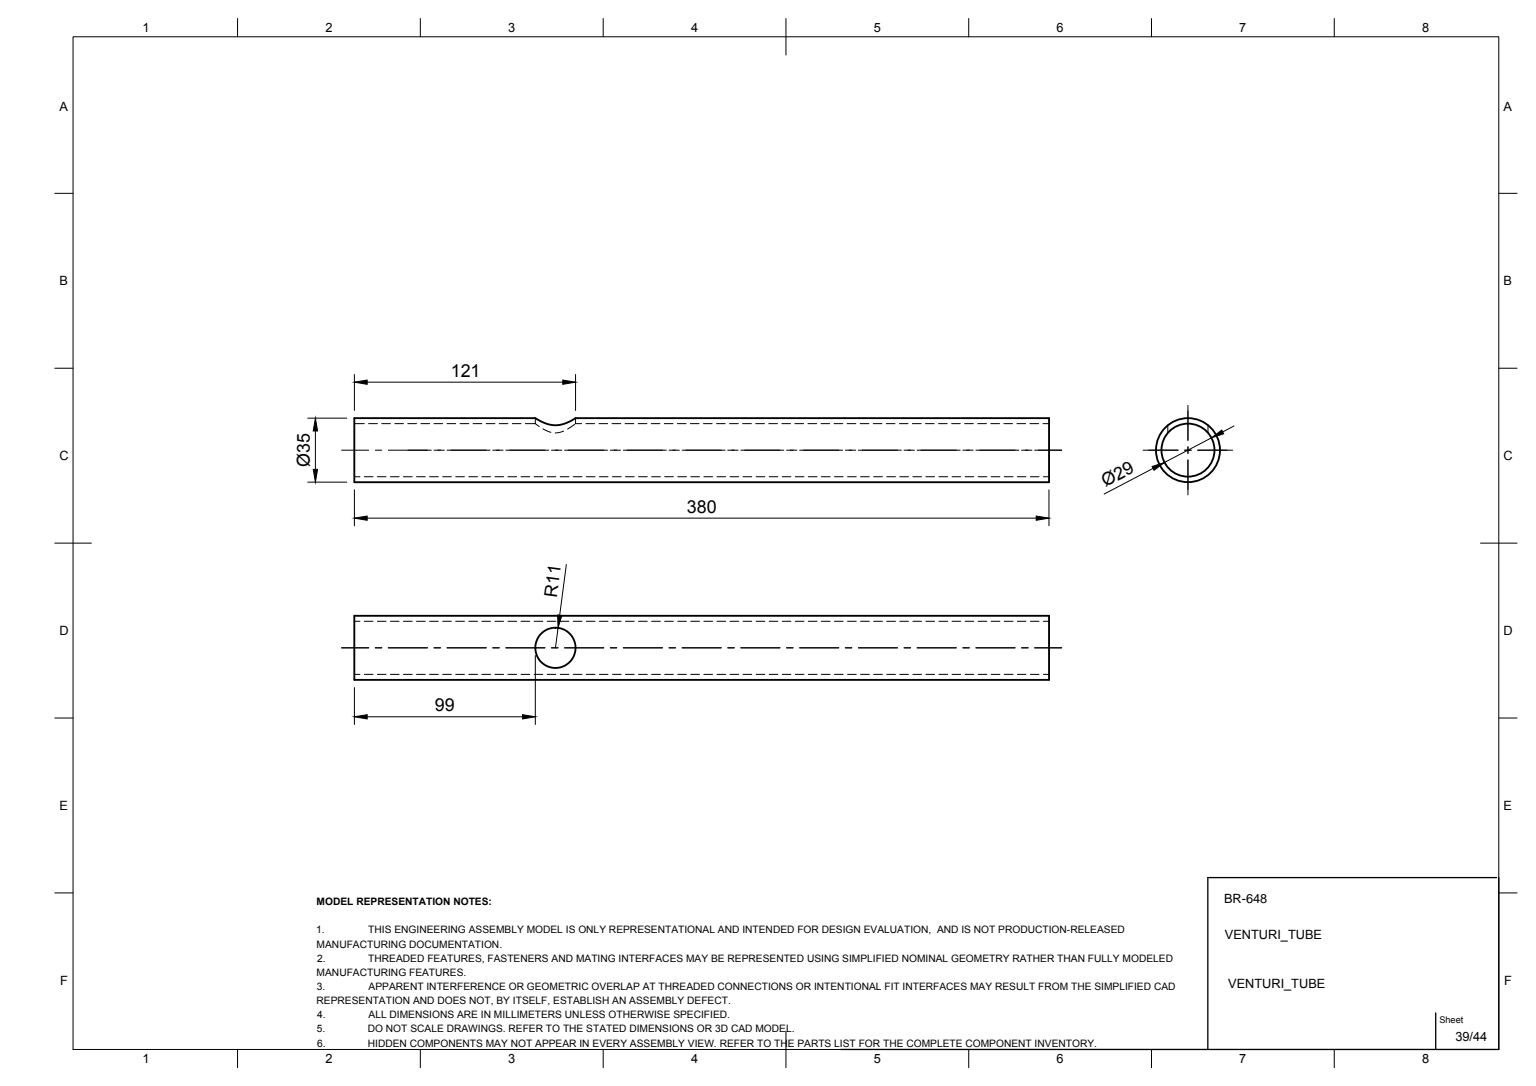
ISO-10303-21;
HEADER;
FILE_DESCRIPTION((''),'2;1');
FILE_NAME('VENTURI_TUBE.step','2026-10-01T22:05:39-07:00',(''),(''),'','','');
FILE_SCHEMA (('AUTOMOTIVE_DESIGN { 1 0 10303 214 3 1 1 }'));
ENDSEC;
DATA;
#10=MECHANICAL_DESIGN_GEOMETRIC_PRESENTATION_REPRESENTATION('',(#635),#24628);
#551=SHAPE_REPRESENTATION_RELATIONSHIP('SRR','None',#24825,#593) ;
#593=ADVANCED_BREP_SHAPE_REPRESENTATION('',(#674),#24615) ;
#635=STYLED_ITEM('',(#25034),#674) ;
#674=MANIFOLD_SOLID_BREP('VENTURI_TUBE',#13177) ;
#908=FACE_BOUND('',#4615,.T.) ;
#909=FACE_BOUND('',#4617,.T.) ;
#985=B_SPLINE_CURVE_WITH_KNOTS('',3,(#23796,#23797,#23798,#23799,#23800,
#23801,#23802,#23803,#23804,#23805,#23806,#23807,#23808,#23809),
 .UNSPECIFIED.,.F.,.F.,(4,2,2,2,2,2,4),(0.,0.222195827909919,0.444391655819838,
0.888783311639677,1.32318070684216,1.54037940444341,1.75757810204465),
 .UNSPECIFIED.) ;
#986=B_SPLINE_CURVE_WITH_KNOTS('',3,(#23811,#23812,#23813,#23814,#23815,
#23816,#23817,#23818,#23819,#23820,#23821,#23822,#23823,#23824),
 .UNSPECIFIED.,.F.,.F.,(4,2,2,2,2,2,4),(5.27273430613395,5.48993300373519,
5.70713170133643,6.14152909653892,6.58592075235876,6.80811658026868,7.0303124081786),
 .UNSPECIFIED.) ;
#987=B_SPLINE_CURVE_WITH_KNOTS('',3,(#23828,#23829,#23830,#23831,#23832,
#23833,#23834,#23835,#23836,#23837,#23838,#23839,#23840,#23841),
 .UNSPECIFIED.,.F.,.F.,(4,2,2,2,2,2,4),(0.,0.215433509152083,0.430867018304165,
0.86173403660833,1.28909704518263,1.50277854946978,1.71646005375693),
 .UNSPECIFIED.) ;
#988=B_SPLINE_CURVE_WITH_KNOTS('',3,(#23843,#23844,#23845,#23846,#23847,
#23848,#23849,#23850,#23851,#23852,#23853,#23854,#23855,#23856),
 .UNSPECIFIED.,.F.,.F.,(4,2,2,2,2,2,4),(5.14938016127078,5.36306166555793,
5.57674316984508,6.00410617841938,6.43497319672355,6.65040670587563,6.86584021502771),
 .UNSPECIFIED.) ;
#989=B_SPLINE_CURVE_WITH_KNOTS('',3,(#23857,#23858,#23859,#23860,#23861,
#23862,#23863,#23864,#23865,#23866,#23867,#23868,#23869,#23870,#23871,#23872,
#23873,#23874,#23875,#23876,#23877,#23878,#23879,#23880,#23881,#23882),
 .UNSPECIFIED.,.F.,.F.,(4,2,2,2,2,2,2,2,2,2,2,2,4),(1.71646005375693,1.93014155804408,
2.14382306233123,2.57118607090553,3.00205308920969,3.21748659836177,3.43292010751385,
3.64835361666594,3.86378712581802,4.29465414412218,4.72201715269648,4.93569865698363,
5.14938016127078),.UNSPECIFIED.) ;
#990=B_SPLINE_CURVE_WITH_KNOTS('',3,(#23883,#23884,#23885,#23886,#23887,
#23888,#23889,#23890,#23891,#23892,#23893,#23894,#23895,#23896,#23897,#23898,
#23899,#23900,#23901,#23902,#23903,#23904,#23905,#23906,#23907,#23908),
 .UNSPECIFIED.,.F.,.F.,(4,2,2,2,2,2,2,2,2,2,2,2,4),(1.75757810204465,1.97477679964589,
2.19197549724714,2.62637289244962,3.07076454826946,3.29296037617938,3.5151562040893,
3.73735203199922,3.95954785990914,4.40393951572897,4.83833691093146,5.0555356085327,
5.27273430613395),.UNSPECIFIED.) ;
#1707=LINE('',#23826,#2543) ;
#1708=LINE('',#23912,#2544) ;
#1709=LINE('',#23914,#2545) ;
#1710=LINE('',#23919,#2546) ;
#1711=LINE('',#23921,#2547) ;
#2543=VECTOR('',#19160,1.1) ;
#2544=VECTOR('',#19165,1.45) ;
#2545=VECTOR('',#19166,1.45) ;
#2546=VECTOR('',#19173,1.75) ;
#2547=VECTOR('',#19174,1.75) ;
#2917=CYLINDRICAL_SURFACE('',#15183,1.1) ;
#2918=CYLINDRICAL_SURFACE('',#15184,1.45) ;
#2919=CYLINDRICAL_SURFACE('',#15187,1.75) ;
#3622=FACE_OUTER_BOUND('',#4611,.T.) ;
#3623=FACE_OUTER_BOUND('',#4612,.T.) ;
#3624=FACE_OUTER_BOUND('',#4613,.T.) ;
#3625=FACE_OUTER_BOUND('',#4614,.T.) ;
#3626=FACE_OUTER_BOUND('',#4616,.T.) ;
#4611=EDGE_LOOP('',(#11567,#11568,#11569,#11570,#11571,#11572,#11573,#11574)) ;
#4612=EDGE_LOOP('',(#11575,#11576,#11577,#11578,#11579,#11580,#11581,#11582,
#11583)) ;
#4613=EDGE_LOOP('',(#11584,#11585,#11586,#11587,#11588,#11589,#11590,#11591,
#11592)) ;
#4614=EDGE_LOOP('',(#11593)) ;
#4615=EDGE_LOOP('',(#11594)) ;
#4616=EDGE_LOOP('',(#11595)) ;
#4617=EDGE_LOOP('',(#11596)) ;
#5469=CIRCLE('',#15185,1.45) ;
#5470=CIRCLE('',#15186,1.45) ;
#5471=CIRCLE('',#15188,1.75) ;
#5472=CIRCLE('',#15189,1.75) ;
#6591=VERTEX_POINT('',#23794) ;
#6592=VERTEX_POINT('',#23795) ;
#6593=VERTEX_POINT('',#23810) ;
#6594=VERTEX_POINT('',#23825) ;
#6595=VERTEX_POINT('',#23827) ;
#6596=VERTEX_POINT('',#23842) ;
#6597=VERTEX_POINT('',#23910) ;
#6598=VERTEX_POINT('',#23913) ;
#6599=VERTEX_POINT('',#23917) ;
#6600=VERTEX_POINT('',#23920) ;
#8273=EDGE_CURVE('',#6591,#6592,#985,.T.) ;
#8274=EDGE_CURVE('',#6593,#6591,#986,.T.) ;
#8275=EDGE_CURVE('',#6593,#6594,#1707,.T.) ;
#8276=EDGE_CURVE('',#6595,#6594,#987,.T.) ;
#8277=EDGE_CURVE('',#6596,#6595,#988,.T.) ;
#8278=EDGE_CURVE('',#6594,#6596,#989,.T.) ;
#8279=EDGE_CURVE('',#6592,#6593,#990,.T.) ;
#8280=EDGE_CURVE('',#6597,#6597,#5469,.T.) ;
#8281=EDGE_CURVE('',#6597,#6593,#1708,.T.) ;
#8282=EDGE_CURVE('',#6592,#6598,#1709,.T.) ;
#8283=EDGE_CURVE('',#6598,#6598,#5470,.T.) ;
#8284=EDGE_CURVE('',#6599,#6599,#5471,.T.) ;
#8285=EDGE_CURVE('',#6599,#6596,#1710,.T.) ;
#8286=EDGE_CURVE('',#6594,#6600,#1711,.T.) ;
#8287=EDGE_CURVE('',#6600,#6600,#5472,.T.) ;
#11567=ORIENTED_EDGE('',*,*,#8273,.F.) ;
#11568=ORIENTED_EDGE('',*,*,#8274,.F.) ;
#11569=ORIENTED_EDGE('',*,*,#8275,.T.) ;
#11570=ORIENTED_EDGE('',*,*,#8276,.F.) ;
#11571=ORIENTED_EDGE('',*,*,#8277,.F.) ;
#11572=ORIENTED_EDGE('',*,*,#8278,.F.) ;
#11573=ORIENTED_EDGE('',*,*,#8275,.F.) ;
#11574=ORIENTED_EDGE('',*,*,#8279,.F.) ;
#11575=ORIENTED_EDGE('',*,*,#8280,.F.) ;
#11576=ORIENTED_EDGE('',*,*,#8281,.T.) ;
#11577=ORIENTED_EDGE('',*,*,#8274,.T.) ;
#11578=ORIENTED_EDGE('',*,*,#8273,.T.) ;
#11579=ORIENTED_EDGE('',*,*,#8282,.T.) ;
#11580=ORIENTED_EDGE('',*,*,#8283,.F.) ;
#11581=ORIENTED_EDGE('',*,*,#8282,.F.) ;
#11582=ORIENTED_EDGE('',*,*,#8279,.T.) ;
#11583=ORIENTED_EDGE('',*,*,#8281,.F.) ;
#11584=ORIENTED_EDGE('',*,*,#8284,.F.) ;
#11585=ORIENTED_EDGE('',*,*,#8285,.T.) ;
#11586=ORIENTED_EDGE('',*,*,#8277,.T.) ;
#11587=ORIENTED_EDGE('',*,*,#8276,.T.) ;
#11588=ORIENTED_EDGE('',*,*,#8286,.T.) ;
#11589=ORIENTED_EDGE('',*,*,#8287,.F.) ;
#11590=ORIENTED_EDGE('',*,*,#8286,.F.) ;
#11591=ORIENTED_EDGE('',*,*,#8278,.T.) ;
#11592=ORIENTED_EDGE('',*,*,#8285,.F.) ;
#11593=ORIENTED_EDGE('',*,*,#8287,.T.) ;
#11594=ORIENTED_EDGE('',*,*,#8280,.T.) ;
#11595=ORIENTED_EDGE('',*,*,#8284,.T.) ;
#11596=ORIENTED_EDGE('',*,*,#8283,.T.) ;
#12287=PLANE('',#15190) ;
#12288=PLANE('',#15191) ;
#13017=ADVANCED_FACE('',(#3622),#2917,.F.) ;
#13018=ADVANCED_FACE('',(#3623),#2918,.F.) ;
#13019=ADVANCED_FACE('',(#3624),#2919,.T.) ;
#13020=ADVANCED_FACE('',(#3625,#908),#12287,.T.) ;
#13021=ADVANCED_FACE('',(#3626,#909),#12288,.T.) ;
#13177=CLOSED_SHELL('',(#13017,#13018,#13019,#13020,#13021)) ;
#15182=AXIS2_PLACEMENT_3D('',#23792,#19156,#19157) ;
#15183=AXIS2_PLACEMENT_3D('',#23793,#19158,#19159) ;
#15184=AXIS2_PLACEMENT_3D('',#23909,#19161,#19162) ;
#15185=AXIS2_PLACEMENT_3D('',#23911,#19163,#19164) ;
#15186=AXIS2_PLACEMENT_3D('',#23915,#19167,#19168) ;
#15187=AXIS2_PLACEMENT_3D('',#23916,#19169,#19170) ;
#15188=AXIS2_PLACEMENT_3D('',#23918,#19171,#19172) ;
#15189=AXIS2_PLACEMENT_3D('',#23922,#19175,#19176) ;
#15190=AXIS2_PLACEMENT_3D('',#23923,#19177,#19178) ;
#15191=AXIS2_PLACEMENT_3D('',#23924,#19179,#19180) ;
#19156=DIRECTION('axis',(0.,0.,1.)) ;
#19157=DIRECTION('refdir',(1.,0.,0.)) ;
#19158=DIRECTION('center_axis',(0.,0.,1.)) ;
#19159=DIRECTION('ref_axis',(1.,0.,0.)) ;
#19160=DIRECTION('',(0.,0.,1.)) ;
#19161=DIRECTION('center_axis',(1.,0.,0.)) ;
#19162=DIRECTION('ref_axis',(0.,0.,-1.)) ;
#19163=DIRECTION('center_axis',(1.,0.,0.)) ;
#19164=DIRECTION('ref_axis',(0.,0.,-1.)) ;
#19165=DIRECTION('',(1.,0.,0.)) ;
#19166=DIRECTION('',(1.,0.,0.)) ;
#19167=DIRECTION('center_axis',(-1.,0.,0.)) ;
#19168=DIRECTION('ref_axis',(0.,0.,-1.)) ;
#19169=DIRECTION('center_axis',(1.,0.,0.)) ;
#19170=DIRECTION('ref_axis',(0.,0.,-1.)) ;
#19171=DIRECTION('center_axis',(1.,0.,0.)) ;
#19172=DIRECTION('ref_axis',(0.,0.,-1.)) ;
#19173=DIRECTION('',(-1.,0.,0.)) ;
#19174=DIRECTION('',(-1.,0.,0.)) ;
#19175=DIRECTION('center_axis',(-1.,0.,0.)) ;
#19176=DIRECTION('ref_axis',(0.,0.,-1.)) ;
#19177=DIRECTION('center_axis',(-1.,0.,0.)) ;
#19178=DIRECTION('ref_axis',(0.,0.,1.)) ;
#19179=DIRECTION('center_axis',(1.,0.,0.)) ;
#19180=DIRECTION('ref_axis',(0.,0.,-1.)) ;
#23792=CARTESIAN_POINT('',(0.,0.,0.)) ;
#23793=CARTESIAN_POINT('Origin',(-3.,-1.8,-15.55)) ;
#23794=CARTESIAN_POINT('',(-3.,-2.9,-15.5552778186154)) ;
#23795=CARTESIAN_POINT('',(-1.9,-1.8,-15.05)) ;
#23796=CARTESIAN_POINT('Ctrl Pts',(-3.,-2.9,-15.5552778186154)) ;
#23797=CARTESIAN_POINT('Ctrl Pts',(-2.92593472403003,-2.9,-15.5552778186154)) ;
#23798=CARTESIAN_POINT('Ctrl Pts',(-2.85172404139738,-2.89244970013866,
-15.5463012974331)) ;
#23799=CARTESIAN_POINT('Ctrl Pts',(-2.70730976928893,-2.86290382536062,
-15.5134793386501)) ;
#23800=CARTESIAN_POINT('Ctrl Pts',(-2.6370687680745,-2.84092482077356,-15.4897837774916)) ;
#23801=CARTESIAN_POINT('Ctrl Pts',(-2.43708115985337,-2.75608431930036,
-15.4070006970031)) ;
#23802=CARTESIAN_POINT('Ctrl Pts',(-2.31772068603768,-2.67335560464808,
-15.3370016719564)) ;
#23803=CARTESIAN_POINT('Ctrl Pts',(-2.12879302508191,-2.48442794369232,
-15.2169163796472)) ;
#23804=CARTESIAN_POINT('Ctrl Pts',(-2.04479613304032,-2.36484101063073,
-15.1570971235734)) ;
#23805=CARTESIAN_POINT('Ctrl Pts',(-1.95889743356179,-2.16258851937244,
-15.0942927158064)) ;
#23806=CARTESIAN_POINT('Ctrl Pts',(-1.93671733228809,-2.09139288005492,
-15.0776864580625)) ;
#23807=CARTESIAN_POINT('Ctrl Pts',(-1.90726216861058,-1.94630062852708,
-15.0555340958438)) ;
#23808=CARTESIAN_POINT('Ctrl Pts',(-1.9,-1.87239956586708,-15.05)) ;
#23809=CARTESIAN_POINT('Ctrl Pts',(-1.9,-1.8,-15.05)) ;
#23810=CARTESIAN_POINT('',(-4.1,-1.8,-15.05)) ;
#23811=CARTESIAN_POINT('Ctrl Pts',(-4.1,-1.8,-15.05)) ;
#23812=CARTESIAN_POINT('Ctrl Pts',(-4.1,-1.87239956586708,-15.05)) ;
#23813=CARTESIAN_POINT('Ctrl Pts',(-4.09273783138942,-1.94630062852708,
-15.0555340958438)) ;
#23814=CARTESIAN_POINT('Ctrl Pts',(-4.06328266771191,-2.09139288005492,
-15.0776864580625)) ;
#23815=CARTESIAN_POINT('Ctrl Pts',(-4.04110256643821,-2.16258851937244,
-15.0942927158064)) ;
#23816=CARTESIAN_POINT('Ctrl Pts',(-3.95520386695968,-2.36484101063073,
-15.1570971235734)) ;
#23817=CARTESIAN_POINT('Ctrl Pts',(-3.87120697491809,-2.48442794369232,
-15.2169163796472)) ;
#23818=CARTESIAN_POINT('Ctrl Pts',(-3.68227931396233,-2.67335560464808,
-15.3370016719564)) ;
#23819=CARTESIAN_POINT('Ctrl Pts',(-3.56291884014663,-2.75608431930036,
-15.4070006970031)) ;
#23820=CARTESIAN_POINT('Ctrl Pts',(-3.3629312319255,-2.84092482077356,-15.4897837774916)) ;
#23821=CARTESIAN_POINT('Ctrl Pts',(-3.29269023071107,-2.86290382536062,
-15.5134793386501)) ;
#23822=CARTESIAN_POINT('Ctrl Pts',(-3.14827595860262,-2.89244970013866,
-15.5463012974331)) ;
#23823=CARTESIAN_POINT('Ctrl Pts',(-3.07406527596997,-2.9,-15.5552778186154)) ;
#23824=CARTESIAN_POINT('Ctrl Pts',(-3.,-2.9,-15.5552778186154)) ;
#23825=CARTESIAN_POINT('',(-4.1,-1.8,-14.75)) ;
#23826=CARTESIAN_POINT('',(-4.1,-1.8,-15.55)) ;
#23827=CARTESIAN_POINT('',(-3.,-2.9,-15.1389342411184)) ;
#23828=CARTESIAN_POINT('Ctrl Pts',(-3.,-2.9,-15.1389342411184)) ;
#23829=CARTESIAN_POINT('Ctrl Pts',(-3.07181116971736,-2.9,-15.1389342411184)) ;
#23830=CARTESIAN_POINT('Ctrl Pts',(-3.14499752680644,-2.89286661726534,
-15.1330764609861)) ;
#23831=CARTESIAN_POINT('Ctrl Pts',(-3.28883700701042,-2.86393369738317,
-15.1104380225034)) ;
#23832=CARTESIAN_POINT('Ctrl Pts',(-3.3595029893093,-2.84215035317734,-15.0937184190741)) ;
#23833=CARTESIAN_POINT('Ctrl Pts',(-3.56118090687537,-2.75726493295417,
-15.0333835136228)) ;
#23834=CARTESIAN_POINT('Ctrl Pts',(-3.68198795957211,-2.6736469590383,-14.9799062284422)) ;
#23835=CARTESIAN_POINT('Ctrl Pts',(-3.87286762925623,-2.48276728935417,
-14.8851973706734)) ;
#23836=CARTESIAN_POINT('Ctrl Pts',(-3.95701740777658,-2.36176319521959,
-14.8367787014793)) ;
#23837=CARTESIAN_POINT('Ctrl Pts',(-4.0422651124962,-2.15923323536895,-14.7858537872249)) ;
#23838=CARTESIAN_POINT('Ctrl Pts',(-4.06409704750744,-2.08825332179439,
-14.7723789472322)) ;
#23839=CARTESIAN_POINT('Ctrl Pts',(-4.09297019244892,-1.9442520796829,-14.7544468449727)) ;
#23840=CARTESIAN_POINT('Ctrl Pts',(-4.1,-1.87122716809572,-14.75)) ;
#23841=CARTESIAN_POINT('Ctrl Pts',(-4.1,-1.8,-14.75)) ;
#23842=CARTESIAN_POINT('',(-1.9,-1.8,-14.75)) ;
#23843=CARTESIAN_POINT('Ctrl Pts',(-1.9,-1.8,-14.75)) ;
#23844=CARTESIAN_POINT('Ctrl Pts',(-1.9,-1.87122716809572,-14.75)) ;
#23845=CARTESIAN_POINT('Ctrl Pts',(-1.90702980755108,-1.9442520796829,-14.7544468449727)) ;
#23846=CARTESIAN_POINT('Ctrl Pts',(-1.93590295249256,-2.08825332179439,
-14.7723789472322)) ;
#23847=CARTESIAN_POINT('Ctrl Pts',(-1.9577348875038,-2.15923323536894,-14.7858537872249)) ;
#23848=CARTESIAN_POINT('Ctrl Pts',(-2.04298259222342,-2.36176319521959,
-14.8367787014793)) ;
#23849=CARTESIAN_POINT('Ctrl Pts',(-2.12713237074377,-2.48276728935417,
-14.8851973706734)) ;
#23850=CARTESIAN_POINT('Ctrl Pts',(-2.31801204042789,-2.6736469590383,-14.9799062284422)) ;
#23851=CARTESIAN_POINT('Ctrl Pts',(-2.43881909312463,-2.75726493295417,
-15.0333835136228)) ;
#23852=CARTESIAN_POINT('Ctrl Pts',(-2.6404970106907,-2.84215035317734,-15.0937184190741)) ;
#23853=CARTESIAN_POINT('Ctrl Pts',(-2.71116299298958,-2.86393369738317,
-15.1104380225034)) ;
#23854=CARTESIAN_POINT('Ctrl Pts',(-2.85500247319356,-2.89286661726534,
-15.1330764609861)) ;
#23855=CARTESIAN_POINT('Ctrl Pts',(-2.92818883028264,-2.9,-15.1389342411184)) ;
#23856=CARTESIAN_POINT('Ctrl Pts',(-3.,-2.9,-15.1389342411184)) ;
#23857=CARTESIAN_POINT('Ctrl Pts',(-4.1,-1.8,-14.75)) ;
#23858=CARTESIAN_POINT('Ctrl Pts',(-4.1,-1.72877283190428,-14.75)) ;
#23859=CARTESIAN_POINT('Ctrl Pts',(-4.09297019244892,-1.6557479203171,-14.7544468449727)) ;
#23860=CARTESIAN_POINT('Ctrl Pts',(-4.06409704750744,-1.51174667820561,
-14.7723789472322)) ;
#23861=CARTESIAN_POINT('Ctrl Pts',(-4.0422651124962,-1.44076676463106,-14.7858537872249)) ;
#23862=CARTESIAN_POINT('Ctrl Pts',(-3.95701740777658,-1.23823680478041,
-14.8367787014793)) ;
#23863=CARTESIAN_POINT('Ctrl Pts',(-3.87286762925623,-1.11723271064583,
-14.8851973706734)) ;
#23864=CARTESIAN_POINT('Ctrl Pts',(-3.68198795957211,-0.926353040961702,
-14.9799062284422)) ;
#23865=CARTESIAN_POINT('Ctrl Pts',(-3.56118090687537,-0.842735067045828,
-15.0333835136228)) ;
#23866=CARTESIAN_POINT('Ctrl Pts',(-3.3595029893093,-0.757849646822659,
-15.0937184190741)) ;
#23867=CARTESIAN_POINT('Ctrl Pts',(-3.28883700701042,-0.736066302616833,
-15.1104380225034)) ;
#23868=CARTESIAN_POINT('Ctrl Pts',(-3.14499752680644,-0.707133382734658,
-15.1330764609861)) ;
#23869=CARTESIAN_POINT('Ctrl Pts',(-3.07181116971736,-0.7,-15.1389342411184)) ;
#23870=CARTESIAN_POINT('Ctrl Pts',(-2.92818883028264,-0.7,-15.1389342411184)) ;
#23871=CARTESIAN_POINT('Ctrl Pts',(-2.85500247319356,-0.707133382734658,
-15.1330764609861)) ;
#23872=CARTESIAN_POINT('Ctrl Pts',(-2.71116299298958,-0.736066302616833,
-15.1104380225034)) ;
#23873=CARTESIAN_POINT('Ctrl Pts',(-2.6404970106907,-0.75784964682266,-15.0937184190741)) ;
#23874=CARTESIAN_POINT('Ctrl Pts',(-2.43881909312463,-0.842735067045828,
-15.0333835136228)) ;
#23875=CARTESIAN_POINT('Ctrl Pts',(-2.31801204042789,-0.926353040961702,
-14.9799062284422)) ;
#23876=CARTESIAN_POINT('Ctrl Pts',(-2.12713237074376,-1.11723271064583,
-14.8851973706734)) ;
#23877=CARTESIAN_POINT('Ctrl Pts',(-2.04298259222342,-1.23823680478041,
-14.8367787014793)) ;
#23878=CARTESIAN_POINT('Ctrl Pts',(-1.9577348875038,-1.44076676463106,-14.7858537872249)) ;
#23879=CARTESIAN_POINT('Ctrl Pts',(-1.93590295249256,-1.51174667820561,
-14.7723789472322)) ;
#23880=CARTESIAN_POINT('Ctrl Pts',(-1.90702980755108,-1.6557479203171,-14.7544468449727)) ;
#23881=CARTESIAN_POINT('Ctrl Pts',(-1.9,-1.72877283190428,-14.75)) ;
#23882=CARTESIAN_POINT('Ctrl Pts',(-1.9,-1.8,-14.75)) ;
#23883=CARTESIAN_POINT('Ctrl Pts',(-1.9,-1.8,-15.05)) ;
#23884=CARTESIAN_POINT('Ctrl Pts',(-1.9,-1.72760043413292,-15.05)) ;
#23885=CARTESIAN_POINT('Ctrl Pts',(-1.90726216861058,-1.65369937147292,
-15.0555340958438)) ;
#23886=CARTESIAN_POINT('Ctrl Pts',(-1.93671733228809,-1.50860711994508,
-15.0776864580625)) ;
#23887=CARTESIAN_POINT('Ctrl Pts',(-1.95889743356178,-1.43741148062756,
-15.0942927158064)) ;
#23888=CARTESIAN_POINT('Ctrl Pts',(-2.04479613304032,-1.23515898936927,
-15.1570971235734)) ;
#23889=CARTESIAN_POINT('Ctrl Pts',(-2.12879302508191,-1.11557205630768,
-15.2169163796472)) ;
#23890=CARTESIAN_POINT('Ctrl Pts',(-2.31772068603768,-0.92664439535192,
-15.3370016719564)) ;
#23891=CARTESIAN_POINT('Ctrl Pts',(-2.43708115985337,-0.843915680699641,
-15.4070006970031)) ;
#23892=CARTESIAN_POINT('Ctrl Pts',(-2.6370687680745,-0.759075179226438,
-15.4897837774916)) ;
#23893=CARTESIAN_POINT('Ctrl Pts',(-2.70730976928893,-0.737096174639381,
-15.5134793386501)) ;
#23894=CARTESIAN_POINT('Ctrl Pts',(-2.85172404139738,-0.707550299861341,
-15.5463012974331)) ;
#23895=CARTESIAN_POINT('Ctrl Pts',(-2.92593472403003,-0.7,-15.5552778186154)) ;
#23896=CARTESIAN_POINT('Ctrl Pts',(-3.07406527596997,-0.7,-15.5552778186154)) ;
#23897=CARTESIAN_POINT('Ctrl Pts',(-3.14827595860262,-0.707550299861341,
-15.5463012974331)) ;
#23898=CARTESIAN_POINT('Ctrl Pts',(-3.29269023071107,-0.737096174639381,
-15.5134793386501)) ;
#23899=CARTESIAN_POINT('Ctrl Pts',(-3.3629312319255,-0.759075179226438,
-15.4897837774916)) ;
#23900=CARTESIAN_POINT('Ctrl Pts',(-3.56291884014663,-0.843915680699641,
-15.4070006970031)) ;
#23901=CARTESIAN_POINT('Ctrl Pts',(-3.68227931396233,-0.92664439535192,
-15.3370016719564)) ;
#23902=CARTESIAN_POINT('Ctrl Pts',(-3.87120697491809,-1.11557205630768,
-15.2169163796472)) ;
#23903=CARTESIAN_POINT('Ctrl Pts',(-3.95520386695968,-1.23515898936927,
-15.1570971235734)) ;
#23904=CARTESIAN_POINT('Ctrl Pts',(-4.04110256643821,-1.43741148062756,
-15.0942927158064)) ;
#23905=CARTESIAN_POINT('Ctrl Pts',(-4.06328266771191,-1.50860711994508,
-15.0776864580625)) ;
#23906=CARTESIAN_POINT('Ctrl Pts',(-4.09273783138942,-1.65369937147292,
-15.0555340958438)) ;
#23907=CARTESIAN_POINT('Ctrl Pts',(-4.1,-1.72760043413292,-15.05)) ;
#23908=CARTESIAN_POINT('Ctrl Pts',(-4.1,-1.8,-15.05)) ;
#23909=CARTESIAN_POINT('Origin',(-11.,-1.8,-16.5)) ;
#23910=CARTESIAN_POINT('',(-30.,-1.8,-15.05)) ;
#23911=CARTESIAN_POINT('Origin',(-30.,-1.8,-16.5)) ;
#23912=CARTESIAN_POINT('',(-11.,-1.8,-15.05)) ;
#23913=CARTESIAN_POINT('',(8.,-1.8,-15.05)) ;
#23914=CARTESIAN_POINT('',(-11.,-1.8,-15.05)) ;
#23915=CARTESIAN_POINT('Origin',(8.,-1.8,-16.5)) ;
#23916=CARTESIAN_POINT('Origin',(-11.,-1.8,-16.5)) ;
#23917=CARTESIAN_POINT('',(8.,-1.8,-14.75)) ;
#23918=CARTESIAN_POINT('Origin',(8.,-1.8,-16.5)) ;
#23919=CARTESIAN_POINT('',(-11.,-1.8,-14.75)) ;
#23920=CARTESIAN_POINT('',(-30.,-1.8,-14.75)) ;
#23921=CARTESIAN_POINT('',(-11.,-1.8,-14.75)) ;
#23922=CARTESIAN_POINT('Origin',(-30.,-1.8,-16.5)) ;
#23923=CARTESIAN_POINT('Origin',(-30.,-1.8,-16.5)) ;
#23924=CARTESIAN_POINT('Origin',(8.,-1.8,-16.5)) ;
#24567=UNCERTAINTY_MEASURE_WITH_UNIT(LENGTH_MEASURE(0.001),#24629,
'DISTANCE_ACCURACY_VALUE',
'Maximum model space distance between geometric entities at asserted c
onnectivities') ;
#24580=UNCERTAINTY_MEASURE_WITH_UNIT(LENGTH_MEASURE(0.001),#24629,
'DISTANCE_ACCURACY_VALUE',
'Maximum model space distance between geometric entities at asserted c
onnectivities') ;
#24615=(
GEOMETRIC_REPRESENTATION_CONTEXT(3)
GLOBAL_UNCERTAINTY_ASSIGNED_CONTEXT((#24567))
GLOBAL_UNIT_ASSIGNED_CONTEXT((#24629,#24631,#24632))
REPRESENTATION_CONTEXT('','3D')
) ;
#24628=(
GEOMETRIC_REPRESENTATION_CONTEXT(3)
GLOBAL_UNCERTAINTY_ASSIGNED_CONTEXT((#24580))
GLOBAL_UNIT_ASSIGNED_CONTEXT((#24629,#24631,#24632))
REPRESENTATION_CONTEXT('','3D')
) ;
#24629=(
LENGTH_UNIT()
NAMED_UNIT(*)
SI_UNIT(.CENTI.,.METRE.)
) ;
#24631=(
NAMED_UNIT(*)
PLANE_ANGLE_UNIT()
SI_UNIT($,.RADIAN.)
) ;
#24632=(
NAMED_UNIT(*)
SI_UNIT($,.STERADIAN.)
SOLID_ANGLE_UNIT()
) ;
#24667=SHAPE_DEFINITION_REPRESENTATION(#24748,#24825) ;
#24748=PRODUCT_DEFINITION_SHAPE('',$,#24873) ;
#24825=SHAPE_REPRESENTATION('',(#15182),#24615) ;
#24838=PRODUCT_DEFINITION_CONTEXT('part definition',#24981,'design') ;
#24873=PRODUCT_DEFINITION('VENTURI_TUBE','VENTURI_TUBE',#24920,
#24838) ;
#24920=PRODUCT_DEFINITION_FORMATION('',$,#25017) ;
#24981=APPLICATION_CONTEXT(
'Core Data for Automotive Mechanical Design Process') ;
#24982=PRODUCT_CONTEXT('part definition',#24981,'mechanical') ;
#25017=PRODUCT('VENTURI_TUBE','VENTURI_TUBE',$,(#24982)) ;
#25034=PRESENTATION_STYLE_ASSIGNMENT((#25044)) ;
#25044=SURFACE_STYLE_USAGE(.BOTH.,#25054) ;
#25054=SURFACE_SIDE_STYLE('',(#25064)) ;
#25064=SURFACE_STYLE_FILL_AREA(#25074) ;
#25074=FILL_AREA_STYLE('Stainless Steel - Satin',(#25084)) ;
#25084=FILL_AREA_STYLE_COLOUR('Stainless Steel - Satin',#25094) ;
#25094=COLOUR_RGB('Stainless Steel - Satin', 0.31764706, 0.68627451, 0.89019608) ;
ENDSEC;
END-ISO-10303-21;
